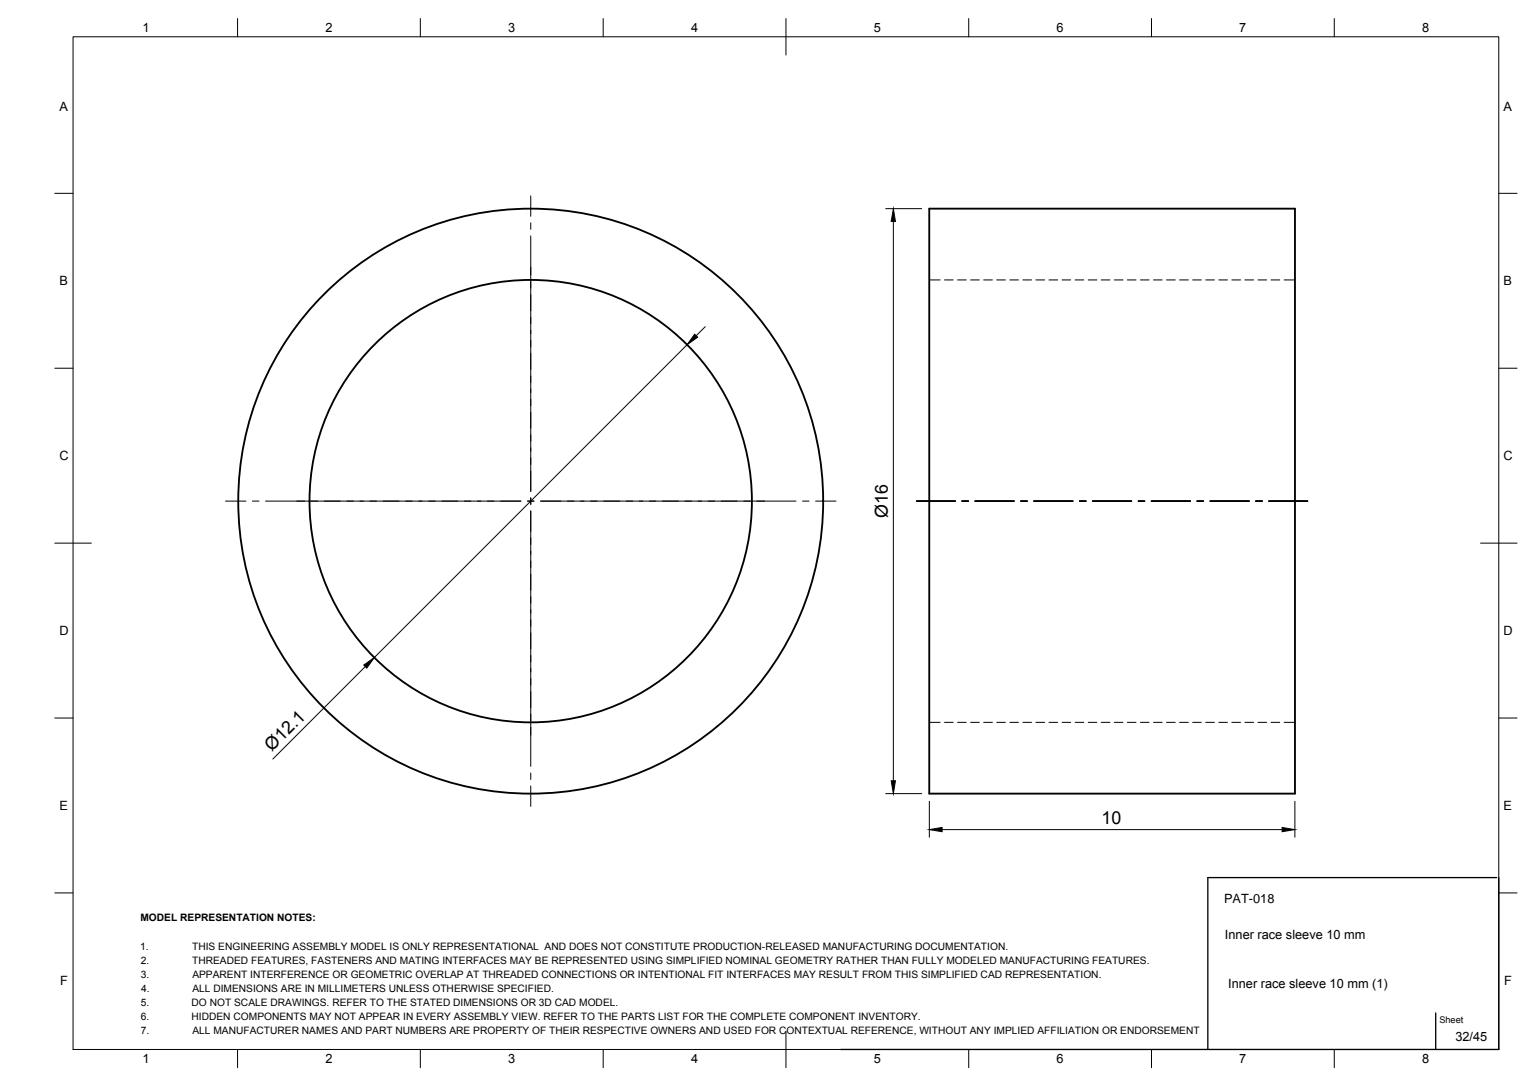
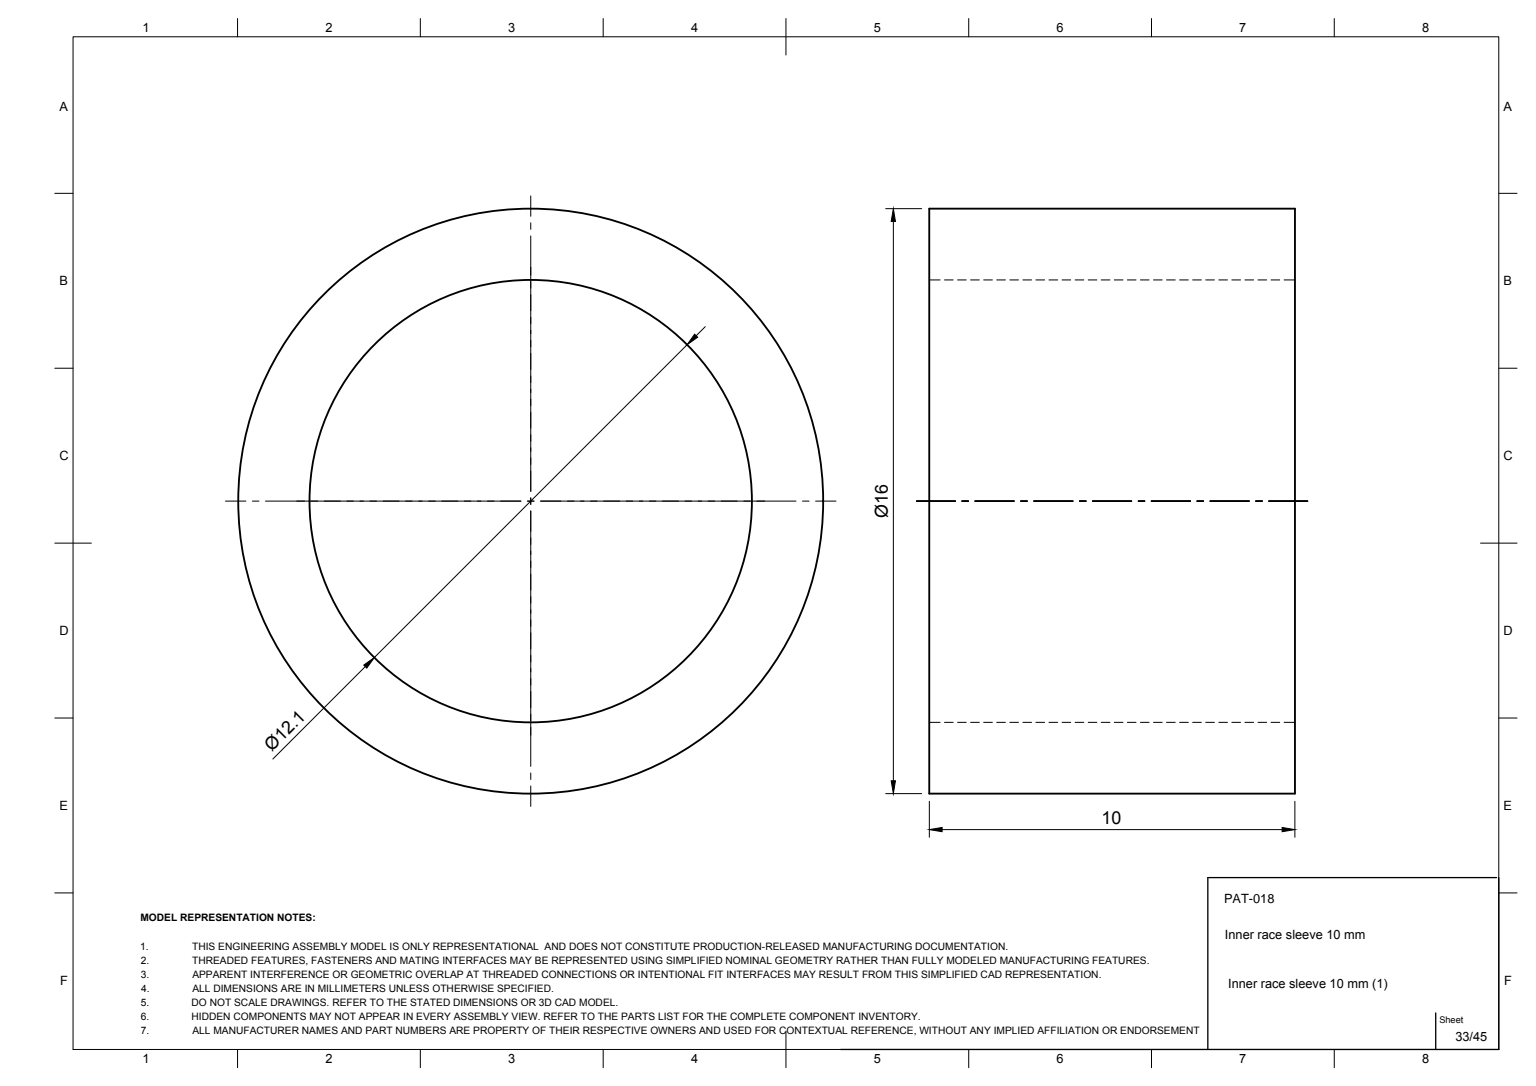
ISO-10303-21;
HEADER;
/* Generated by software containing ST-Developer
 * from STEP Tools, Inc. (www.steptools.com) 
 */

FILE_DESCRIPTION(
/* description */ ('Cam-driven reciprocating slide'),
/* implementation_level */ '2;1');

FILE_NAME(
/* name */ 'Inner race sleeve 10 mm.step',
/* time_stamp */ '2026-10-28T03:25:20-07:00',
/* author */ (''),
/* organization */ (''),
/* preprocessor_version */ 'ST-DEVELOPER v20.2',
/* originating_system */ 'Autodesk Translation Framework v15.17.0.0',
/* authorisation */ '');

FILE_SCHEMA (('AUTOMOTIVE_DESIGN { 1 0 10303 214 3 1 1 }'));
ENDSEC;

DATA;
#10=MECHANICAL_DESIGN_GEOMETRIC_PRESENTATION_REPRESENTATION('',(#452),#13277);
#371=SHAPE_REPRESENTATION_RELATIONSHIP('SRR','None',#13467,#408);
#408=ADVANCED_BREP_SHAPE_REPRESENTATION('',(#494),#13262);
#452=STYLED_ITEM('',(#13720),#494);
#494=MANIFOLD_SOLID_BREP('Body1',#6430);
#644=FACE_BOUND('',#1694,.T.);
#645=FACE_BOUND('',#1696,.T.);
#833=PLANE('',#7420);
#834=PLANE('',#7421);
#1175=FACE_OUTER_BOUND('',#1691,.T.);
#1176=FACE_OUTER_BOUND('',#1692,.T.);
#1177=FACE_OUTER_BOUND('',#1693,.T.);
#1178=FACE_OUTER_BOUND('',#1695,.T.);
#1691=EDGE_LOOP('',(#5492,#5493,#5494,#5495));
#1692=EDGE_LOOP('',(#5496,#5497,#5498,#5499));
#1693=EDGE_LOOP('',(#5500));
#1694=EDGE_LOOP('',(#5501));
#1695=EDGE_LOOP('',(#5502));
#1696=EDGE_LOOP('',(#5503));
#2144=LINE('',#12679,#2583);
#2145=LINE('',#12685,#2584);
#2583=VECTOR('',#9106,0.605);
#2584=VECTOR('',#9113,0.8);
#2963=CIRCLE('',#7415,0.605);
#2964=CIRCLE('',#7416,0.605);
#2965=CIRCLE('',#7418,0.8);
#2966=CIRCLE('',#7419,0.8);
#3426=VERTEX_POINT('',#12676);
#3427=VERTEX_POINT('',#12678);
#3428=VERTEX_POINT('',#12682);
#3429=VERTEX_POINT('',#12684);
#4136=EDGE_CURVE('',#3426,#3426,#2963,.T.);
#4137=EDGE_CURVE('',#3426,#3427,#2144,.T.);
#4138=EDGE_CURVE('',#3427,#3427,#2964,.T.);
#4139=EDGE_CURVE('',#3428,#3428,#2965,.T.);
#4140=EDGE_CURVE('',#3428,#3429,#2145,.T.);
#4141=EDGE_CURVE('',#3429,#3429,#2966,.T.);
#5492=ORIENTED_EDGE('',*,*,#4136,.F.);
#5493=ORIENTED_EDGE('',*,*,#4137,.T.);
#5494=ORIENTED_EDGE('',*,*,#4138,.T.);
#5495=ORIENTED_EDGE('',*,*,#4137,.F.);
#5496=ORIENTED_EDGE('',*,*,#4139,.F.);
#5497=ORIENTED_EDGE('',*,*,#4140,.T.);
#5498=ORIENTED_EDGE('',*,*,#4141,.T.);
#5499=ORIENTED_EDGE('',*,*,#4140,.F.);
#5500=ORIENTED_EDGE('',*,*,#4139,.T.);
#5501=ORIENTED_EDGE('',*,*,#4136,.T.);
#5502=ORIENTED_EDGE('',*,*,#4141,.F.);
#5503=ORIENTED_EDGE('',*,*,#4138,.F.);
#5986=CYLINDRICAL_SURFACE('',#7414,0.605);
#5987=CYLINDRICAL_SURFACE('',#7417,0.8);
#6293=ADVANCED_FACE('',(#1175),#5986,.F.);
#6294=ADVANCED_FACE('',(#1176),#5987,.T.);
#6295=ADVANCED_FACE('',(#1177,#644),#833,.T.);
#6296=ADVANCED_FACE('',(#1178,#645),#834,.F.);
#6430=CLOSED_SHELL('',(#6293,#6294,#6295,#6296));
#7413=AXIS2_PLACEMENT_3D('',#12674,#9100,#9101);
#7414=AXIS2_PLACEMENT_3D('',#12675,#9102,#9103);
#7415=AXIS2_PLACEMENT_3D('',#12677,#9104,#9105);
#7416=AXIS2_PLACEMENT_3D('',#12680,#9107,#9108);
#7417=AXIS2_PLACEMENT_3D('',#12681,#9109,#9110);
#7418=AXIS2_PLACEMENT_3D('',#12683,#9111,#9112);
#7419=AXIS2_PLACEMENT_3D('',#12686,#9114,#9115);
#7420=AXIS2_PLACEMENT_3D('',#12687,#9116,#9117);
#7421=AXIS2_PLACEMENT_3D('',#12688,#9118,#9119);
#9100=DIRECTION('axis',(0.,0.,1.));
#9101=DIRECTION('refdir',(1.,0.,0.));
#9102=DIRECTION('center_axis',(0.,1.,0.));
#9103=DIRECTION('ref_axis',(1.,0.,0.));
#9104=DIRECTION('center_axis',(0.,-1.,0.));
#9105=DIRECTION('ref_axis',(1.,0.,0.));
#9106=DIRECTION('',(0.,-1.,0.));
#9107=DIRECTION('center_axis',(0.,-1.,0.));
#9108=DIRECTION('ref_axis',(1.,0.,0.));
#9109=DIRECTION('center_axis',(0.,1.,0.));
#9110=DIRECTION('ref_axis',(1.,0.,0.));
#9111=DIRECTION('center_axis',(0.,1.,0.));
#9112=DIRECTION('ref_axis',(1.,0.,0.));
#9113=DIRECTION('',(0.,-1.,0.));
#9114=DIRECTION('center_axis',(0.,1.,0.));
#9115=DIRECTION('ref_axis',(1.,0.,0.));
#9116=DIRECTION('center_axis',(0.,1.,0.));
#9117=DIRECTION('ref_axis',(1.,0.,0.));
#9118=DIRECTION('center_axis',(0.,1.,0.));
#9119=DIRECTION('ref_axis',(1.,0.,0.));
#12674=CARTESIAN_POINT('',(0.,0.,0.));
#12675=CARTESIAN_POINT('Origin',(0.,-2.,4.));
#12676=CARTESIAN_POINT('',(-0.605,-1.,4.));
#12677=CARTESIAN_POINT('Origin',(0.,-1.,4.));
#12678=CARTESIAN_POINT('',(-0.605,-2.,4.));
#12679=CARTESIAN_POINT('',(-0.605,-2.,4.));
#12680=CARTESIAN_POINT('Origin',(0.,-2.,4.));
#12681=CARTESIAN_POINT('Origin',(0.,-2.,4.));
#12682=CARTESIAN_POINT('',(-0.8,-1.,4.));
#12683=CARTESIAN_POINT('Origin',(0.,-1.,4.));
#12684=CARTESIAN_POINT('',(-0.8,-2.,4.));
#12685=CARTESIAN_POINT('',(-0.8,-2.,4.));
#12686=CARTESIAN_POINT('Origin',(0.,-2.,4.));
#12687=CARTESIAN_POINT('Origin',(0.,-1.,4.));
#12688=CARTESIAN_POINT('Origin',(0.,-2.,4.));
#13218=UNCERTAINTY_MEASURE_WITH_UNIT(LENGTH_MEASURE(0.001),#13278,
'DISTANCE_ACCURACY_VALUE',
'Maximum model space distance between geometric entities at asserted c
onnectivities');
#13233=UNCERTAINTY_MEASURE_WITH_UNIT(LENGTH_MEASURE(0.001),#13278,
'DISTANCE_ACCURACY_VALUE',
'Maximum model space distance between geometric entities at asserted c
onnectivities');
#13262=(
GEOMETRIC_REPRESENTATION_CONTEXT(3)
GLOBAL_UNCERTAINTY_ASSIGNED_CONTEXT((#13218))
GLOBAL_UNIT_ASSIGNED_CONTEXT((#13278,#13280,#13281))
REPRESENTATION_CONTEXT('','3D')
);
#13277=(
GEOMETRIC_REPRESENTATION_CONTEXT(3)
GLOBAL_UNCERTAINTY_ASSIGNED_CONTEXT((#13233))
GLOBAL_UNIT_ASSIGNED_CONTEXT((#13278,#13280,#13281))
REPRESENTATION_CONTEXT('','3D')
);
#13278=(
LENGTH_UNIT()
NAMED_UNIT(*)
SI_UNIT(.CENTI.,.METRE.)
);
#13280=(
NAMED_UNIT(*)
PLANE_ANGLE_UNIT()
SI_UNIT($,.RADIAN.)
);
#13281=(
NAMED_UNIT(*)
SI_UNIT($,.STERADIAN.)
SOLID_ANGLE_UNIT()
);
#13310=SHAPE_DEFINITION_REPRESENTATION(#13360,#13467);
#13360=PRODUCT_DEFINITION_SHAPE('',$,#13511);
#13467=SHAPE_REPRESENTATION('',(#7413),#13262);
#13482=PRODUCT_DEFINITION_CONTEXT('part definition',#13613,'design');
#13511=PRODUCT_DEFINITION('Inner race sleeve 10 mm',
'Inner race sleeve 10 mm',#13554,#13482);
#13554=PRODUCT_DEFINITION_FORMATION('',$,#13643);
#13613=APPLICATION_CONTEXT(
'Core Data for Automotive Mechanical Design Process');
#13614=PRODUCT_CONTEXT('part definition',#13613,'mechanical');
#13643=PRODUCT('Inner race sleeve 10 mm','Inner race sleeve 10 mm',
'Inner race sleeve 10 mm',(#13614));
#13714=COLOUR_RGB('Grey',0.48,0.52,0.57);
#13715=FILL_AREA_STYLE_COLOUR('',#13714);
#13716=FILL_AREA_STYLE('',(#13715));
#13717=SURFACE_STYLE_FILL_AREA(#13716);
#13718=SURFACE_SIDE_STYLE('',(#13717));
#13719=SURFACE_STYLE_USAGE(.BOTH.,#13718);
#13720=PRESENTATION_STYLE_ASSIGNMENT((#13719));
ENDSEC;
END-ISO-10303-21;
